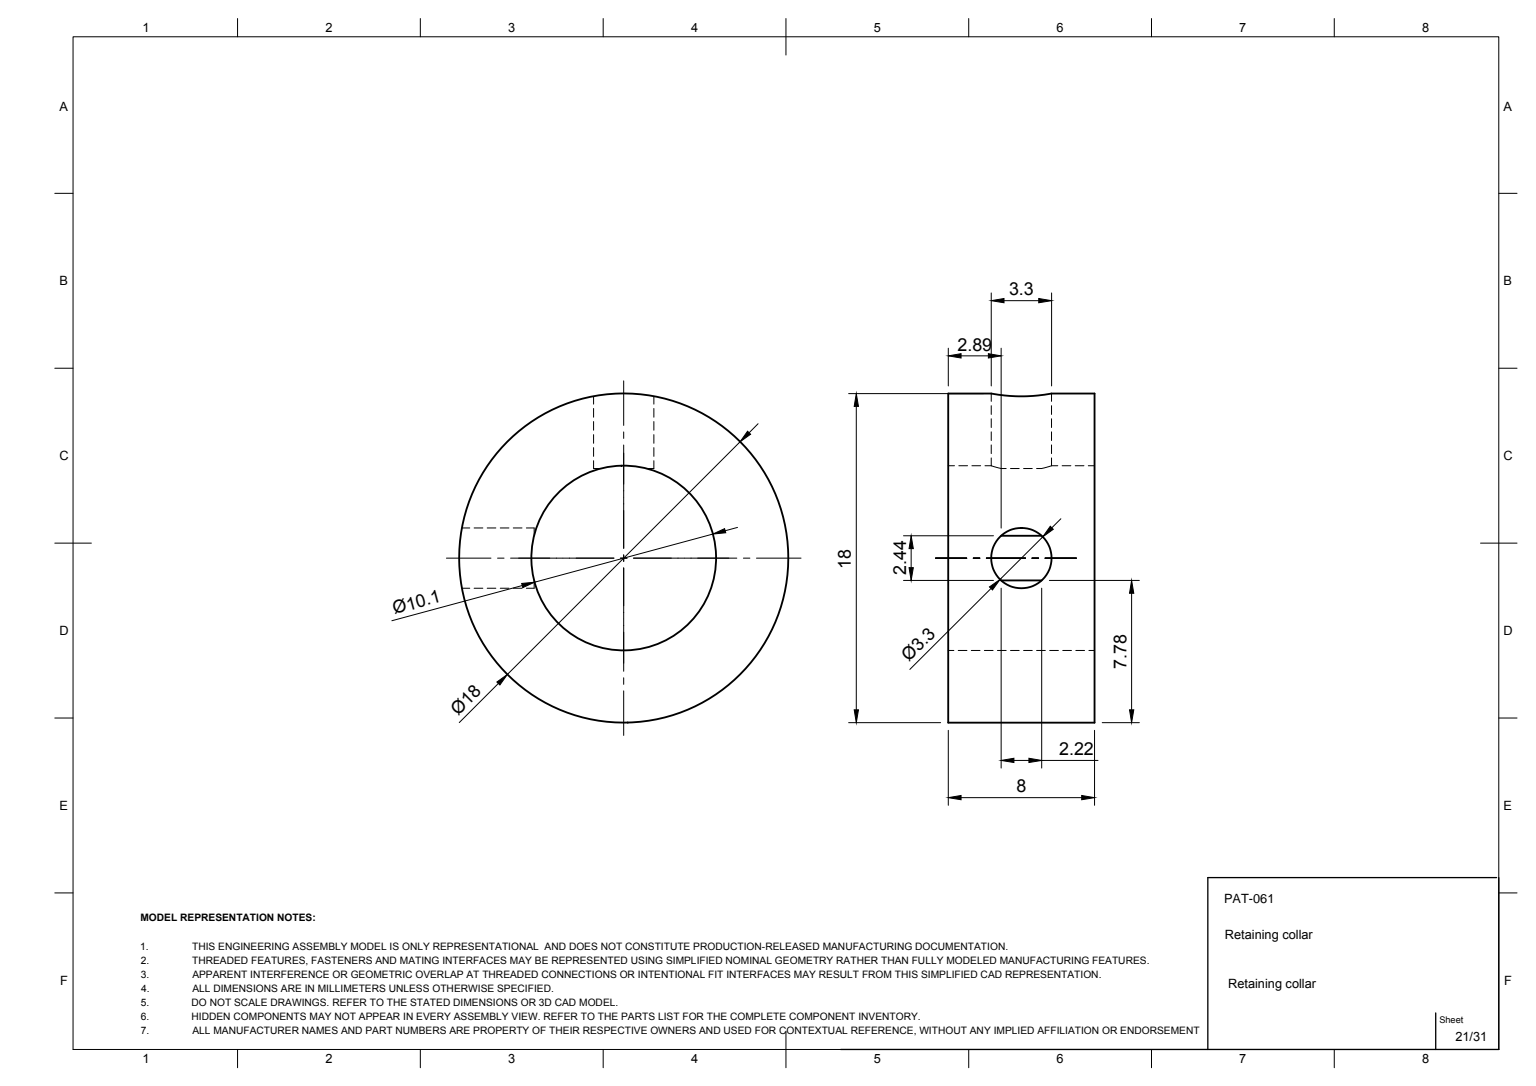
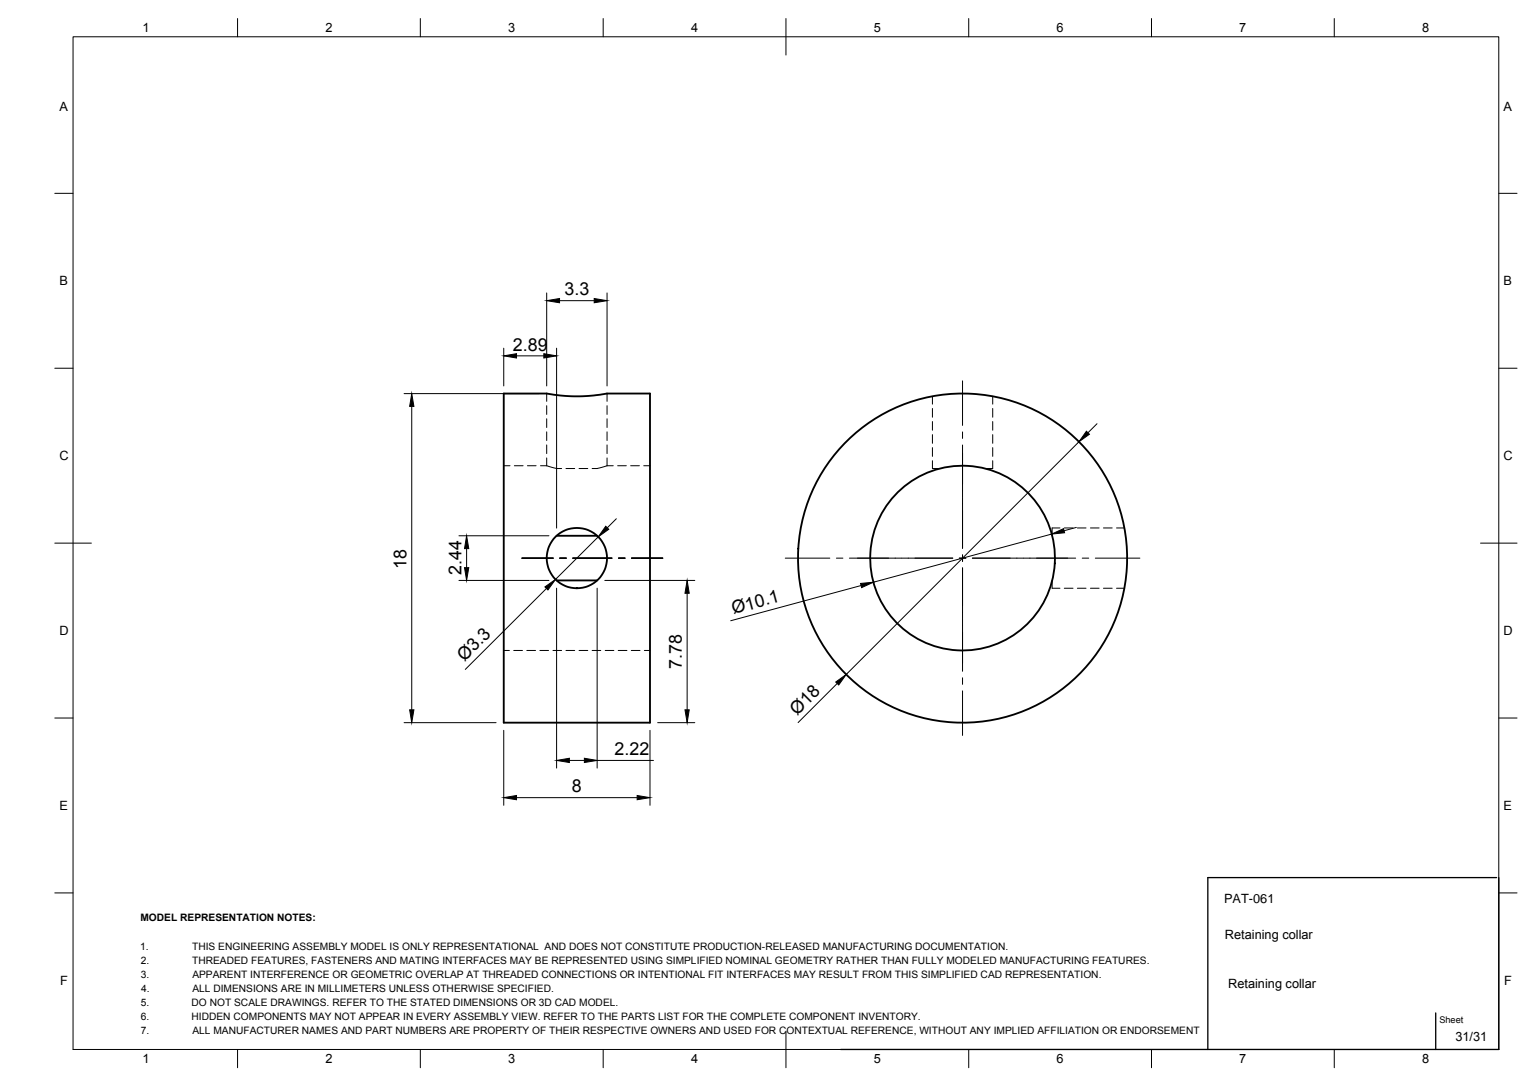
ISO-10303-21;
HEADER;
/* Generated by software containing ST-Developer
 * from STEP Tools, Inc. (www.steptools.com) 
 */

FILE_DESCRIPTION(
/* description */ ('Compact intermittent indexer'),
/* implementation_level */ '2;1');

FILE_NAME(
/* name */ 'Retaining collar.step',
/* time_stamp */ '2026-10-29T16:32:17-07:00',
/* author */ (''),
/* organization */ (''),
/* preprocessor_version */ 'ST-DEVELOPER v20.2',
/* originating_system */ 'Autodesk Translation Framework v15.17.0.0',
/* authorisation */ '');

FILE_SCHEMA (('AUTOMOTIVE_DESIGN { 1 0 10303 214 3 1 1 }'));
ENDSEC;

DATA;
#10=MECHANICAL_DESIGN_GEOMETRIC_PRESENTATION_REPRESENTATION('',(#278),#10837);
#222=SHAPE_REPRESENTATION_RELATIONSHIP('SRR','None',#10958,#246);
#246=ADVANCED_BREP_SHAPE_REPRESENTATION('',(#309),#10825);
#278=STYLED_ITEM('',(#11180),#309);
#309=MANIFOLD_SOLID_BREP('Body1',#5651);
#339=B_SPLINE_CURVE_WITH_KNOTS('',3,(#9829,#9830,#9831,#9832,#9833,#9834,
#9835,#9836,#9837,#9838,#9839,#9840,#9841,#9842,#9843,#9844,#9845,#9846,
#9847,#9848,#9849,#9850,#9851,#9852,#9853,#9854,#9855,#9856,#9857,#9858,
#9859,#9860,#9861,#9862),.UNSPECIFIED.,.T.,.F.,(4,2,2,2,2,2,2,2,2,2,2,2,
2,2,2,2,4),(0.,0.0623062782223143,0.124612556444629,0.186916384615149,0.249220212785669,
0.31152404095619,0.37382786912671,0.436134147349024,0.498440425571339,0.560746703793653,
0.623052982015967,0.685356810186488,0.747660638357008,0.809964466527529,
0.872268294698049,0.934574572920363,0.996880851142677),.UNSPECIFIED.);
#340=B_SPLINE_CURVE_WITH_KNOTS('',3,(#9865,#9866,#9867,#9868,#9869,#9870,
#9871,#9872,#9873,#9874,#9875,#9876,#9877,#9878),.UNSPECIFIED.,.F.,.F.,
(4,2,2,2,2,2,4),(0.618551524396292,0.626563103102765,0.689203386094988,
0.751843669087211,0.814483952079434,0.877124235071657,0.88513581377813),
 .UNSPECIFIED.);
#341=B_SPLINE_CURVE_WITH_KNOTS('',3,(#9881,#9882,#9883,#9884,#9885,#9886,
#9887,#9888,#9889,#9890,#9891,#9892,#9893,#9894),.UNSPECIFIED.,.F.,.F.,
(4,2,2,2,2,2,4),(0.117322411671485,0.125333990377958,0.187974273370181,
0.250614556362404,0.313254839354627,0.37589512234685,0.383906701053323),
 .UNSPECIFIED.);
#342=B_SPLINE_CURVE_WITH_KNOTS('',3,(#9905,#9906,#9907,#9908,#9909,#9910,
#9911,#9912,#9913,#9914),.UNSPECIFIED.,.F.,.F.,(4,2,2,2,4),(0.,0.0623062782223142,
0.124612556444628,0.186916384615149,0.249220212785669),.UNSPECIFIED.);
#343=B_SPLINE_CURVE_WITH_KNOTS('',3,(#9916,#9917,#9918,#9919,#9920,#9921,
#9922,#9923,#9924,#9925),.UNSPECIFIED.,.F.,.F.,(4,2,2,2,4),(0.747660638357008,
0.809964466527529,0.872268294698049,0.934574572920363,0.996880851142677),
 .UNSPECIFIED.);
#344=B_SPLINE_CURVE_WITH_KNOTS('',3,(#9926,#9927,#9928,#9929,#9930,#9931,
#9932,#9933,#9934,#9935,#9936,#9937,#9938,#9939,#9940,#9941,#9942,#9943),
 .UNSPECIFIED.,.F.,.F.,(4,2,2,2,2,2,2,2,4),(0.249220212785669,0.31152404095619,
0.37382786912671,0.436134147349024,0.498440425571339,0.560746703793653,
0.623052982015967,0.685356810186488,0.747660638357008),.UNSPECIFIED.);
#345=B_SPLINE_CURVE_WITH_KNOTS('',3,(#9947,#9948,#9949,#9950,#9951,#9952,
#9953,#9954),.UNSPECIFIED.,.F.,.F.,(4,2,2,4),(0.618551524396292,0.626563103102765,
0.689203386094988,0.751843669087211),.UNSPECIFIED.);
#346=B_SPLINE_CURVE_WITH_KNOTS('',3,(#9958,#9959,#9960,#9961,#9962,#9963,
#9964,#9965),.UNSPECIFIED.,.F.,.F.,(4,2,2,4),(0.250614556362404,0.313254839354627,
0.37589512234685,0.383906701053323),.UNSPECIFIED.);
#347=B_SPLINE_CURVE_WITH_KNOTS('',3,(#9966,#9967,#9968,#9969,#9970,#9971,
#9972,#9973),.UNSPECIFIED.,.F.,.F.,(4,2,2,4),(0.117322411671484,0.125333990377958,
0.187974273370181,0.250614556362404),.UNSPECIFIED.);
#348=B_SPLINE_CURVE_WITH_KNOTS('',3,(#9974,#9975,#9976,#9977,#9978,#9979,
#9980,#9981),.UNSPECIFIED.,.F.,.F.,(4,2,2,4),(0.751843669087211,0.814483952079434,
0.877124235071657,0.885135813778131),.UNSPECIFIED.);
#440=FACE_BOUND('',#1274,.T.);
#441=FACE_BOUND('',#1276,.T.);
#442=FACE_BOUND('',#1278,.T.);
#443=FACE_BOUND('',#1280,.T.);
#569=PLANE('',#6369);
#570=PLANE('',#6374);
#571=PLANE('',#6375);
#572=PLANE('',#6379);
#573=PLANE('',#6386);
#574=PLANE('',#6387);
#852=FACE_OUTER_BOUND('',#1267,.T.);
#853=FACE_OUTER_BOUND('',#1268,.T.);
#854=FACE_OUTER_BOUND('',#1269,.T.);
#855=FACE_OUTER_BOUND('',#1270,.T.);
#856=FACE_OUTER_BOUND('',#1271,.T.);
#857=FACE_OUTER_BOUND('',#1272,.T.);
#858=FACE_OUTER_BOUND('',#1273,.T.);
#859=FACE_OUTER_BOUND('',#1275,.T.);
#860=FACE_OUTER_BOUND('',#1277,.T.);
#861=FACE_OUTER_BOUND('',#1279,.T.);
#1267=EDGE_LOOP('',(#4530,#4531,#4532));
#1268=EDGE_LOOP('',(#4533,#4534,#4535,#4536,#4537,#4538,#4539,#4540));
#1269=EDGE_LOOP('',(#4541,#4542));
#1270=EDGE_LOOP('',(#4543,#4544));
#1271=EDGE_LOOP('',(#4545,#4546,#4547,#4548,#4549,#4550,#4551,#4552,#4553,
#4554,#4555));
#1272=EDGE_LOOP('',(#4556,#4557));
#1273=EDGE_LOOP('',(#4558,#4559,#4560,#4561,#4562,#4563,#4564,#4565,#4566,
#4567,#4568,#4569));
#1274=EDGE_LOOP('',(#4570,#4571,#4572,#4573));
#1275=EDGE_LOOP('',(#4574,#4575,#4576,#4577,#4578,#4579,#4580,#4581,#4582));
#1276=EDGE_LOOP('',(#4583));
#1277=EDGE_LOOP('',(#4584));
#1278=EDGE_LOOP('',(#4585));
#1279=EDGE_LOOP('',(#4586));
#1280=EDGE_LOOP('',(#4587));
#1605=LINE('',#9823,#1963);
#1606=LINE('',#9863,#1964);
#1607=LINE('',#9896,#1965);
#1608=LINE('',#9900,#1966);
#1609=LINE('',#9945,#1967);
#1610=LINE('',#9983,#1968);
#1611=LINE('',#9987,#1969);
#1612=LINE('',#9989,#1970);
#1613=LINE('',#9994,#1971);
#1614=LINE('',#9996,#1972);
#1963=VECTOR('',#7723,1.);
#1964=VECTOR('',#7730,0.165);
#1965=VECTOR('',#7735,1.);
#1966=VECTOR('',#7738,1.);
#1967=VECTOR('',#7743,0.165);
#1968=VECTOR('',#7748,1.);
#1969=VECTOR('',#7753,0.505);
#1970=VECTOR('',#7754,0.505);
#1971=VECTOR('',#7761,0.9);
#1972=VECTOR('',#7762,0.9);
#2366=CIRCLE('',#6370,0.165);
#2367=CIRCLE('',#6371,0.165);
#2368=CIRCLE('',#6373,0.165);
#2369=CIRCLE('',#6376,0.165);
#2370=CIRCLE('',#6378,0.165);
#2371=CIRCLE('',#6381,0.505);
#2372=CIRCLE('',#6382,0.505);
#2373=CIRCLE('',#6384,0.9);
#2374=CIRCLE('',#6385,0.9);
#2764=VERTEX_POINT('',#9821);
#2765=VERTEX_POINT('',#9822);
#2766=VERTEX_POINT('',#9824);
#2767=VERTEX_POINT('',#9828);
#2768=VERTEX_POINT('',#9864);
#2769=VERTEX_POINT('',#9879);
#2770=VERTEX_POINT('',#9898);
#2771=VERTEX_POINT('',#9899);
#2772=VERTEX_POINT('',#9903);
#2773=VERTEX_POINT('',#9904);
#2774=VERTEX_POINT('',#9915);
#2775=VERTEX_POINT('',#9944);
#2776=VERTEX_POINT('',#9946);
#2777=VERTEX_POINT('',#9955);
#2778=VERTEX_POINT('',#9957);
#2779=VERTEX_POINT('',#9985);
#2780=VERTEX_POINT('',#9988);
#2781=VERTEX_POINT('',#9992);
#2782=VERTEX_POINT('',#9995);
#3387=EDGE_CURVE('',#2764,#2765,#1605,.T.);
#3388=EDGE_CURVE('',#2766,#2764,#2366,.T.);
#3389=EDGE_CURVE('',#2765,#2766,#2367,.T.);
#3390=EDGE_CURVE('',#2767,#2767,#339,.T.);
#3391=EDGE_CURVE('',#2767,#2766,#1606,.T.);
#3392=EDGE_CURVE('',#2768,#2764,#340,.T.);
#3393=EDGE_CURVE('',#2768,#2769,#2368,.T.);
#3394=EDGE_CURVE('',#2765,#2769,#341,.T.);
#3395=EDGE_CURVE('',#2769,#2768,#1607,.T.);
#3396=EDGE_CURVE('',#2770,#2771,#1608,.T.);
#3397=EDGE_CURVE('',#2771,#2770,#2369,.T.);
#3398=EDGE_CURVE('',#2772,#2773,#342,.T.);
#3399=EDGE_CURVE('',#2774,#2772,#343,.T.);
#3400=EDGE_CURVE('',#2773,#2774,#344,.T.);
#3401=EDGE_CURVE('',#2773,#2775,#1609,.T.);
#3402=EDGE_CURVE('',#2776,#2775,#345,.T.);
#3403=EDGE_CURVE('',#2776,#2777,#2370,.T.);
#3404=EDGE_CURVE('',#2778,#2777,#346,.T.);
#3405=EDGE_CURVE('',#2771,#2778,#347,.T.);
#3406=EDGE_CURVE('',#2775,#2770,#348,.T.);
#3407=EDGE_CURVE('',#2777,#2776,#1610,.T.);
#3408=EDGE_CURVE('',#2779,#2779,#2371,.T.);
#3409=EDGE_CURVE('',#2779,#2775,#1611,.T.);
#3410=EDGE_CURVE('',#2778,#2780,#1612,.T.);
#3411=EDGE_CURVE('',#2780,#2780,#2372,.T.);
#3412=EDGE_CURVE('',#2781,#2781,#2373,.T.);
#3413=EDGE_CURVE('',#2781,#2773,#1613,.T.);
#3414=EDGE_CURVE('',#2774,#2782,#1614,.T.);
#3415=EDGE_CURVE('',#2782,#2782,#2374,.T.);
#4530=ORIENTED_EDGE('',*,*,#3387,.F.);
#4531=ORIENTED_EDGE('',*,*,#3388,.F.);
#4532=ORIENTED_EDGE('',*,*,#3389,.F.);
#4533=ORIENTED_EDGE('',*,*,#3390,.F.);
#4534=ORIENTED_EDGE('',*,*,#3391,.T.);
#4535=ORIENTED_EDGE('',*,*,#3388,.T.);
#4536=ORIENTED_EDGE('',*,*,#3392,.F.);
#4537=ORIENTED_EDGE('',*,*,#3393,.T.);
#4538=ORIENTED_EDGE('',*,*,#3394,.F.);
#4539=ORIENTED_EDGE('',*,*,#3389,.T.);
#4540=ORIENTED_EDGE('',*,*,#3391,.F.);
#4541=ORIENTED_EDGE('',*,*,#3395,.F.);
#4542=ORIENTED_EDGE('',*,*,#3393,.F.);
#4543=ORIENTED_EDGE('',*,*,#3396,.F.);
#4544=ORIENTED_EDGE('',*,*,#3397,.F.);
#4545=ORIENTED_EDGE('',*,*,#3398,.F.);
#4546=ORIENTED_EDGE('',*,*,#3399,.F.);
#4547=ORIENTED_EDGE('',*,*,#3400,.F.);
#4548=ORIENTED_EDGE('',*,*,#3401,.T.);
#4549=ORIENTED_EDGE('',*,*,#3402,.F.);
#4550=ORIENTED_EDGE('',*,*,#3403,.T.);
#4551=ORIENTED_EDGE('',*,*,#3404,.F.);
#4552=ORIENTED_EDGE('',*,*,#3405,.F.);
#4553=ORIENTED_EDGE('',*,*,#3397,.T.);
#4554=ORIENTED_EDGE('',*,*,#3406,.F.);
#4555=ORIENTED_EDGE('',*,*,#3401,.F.);
#4556=ORIENTED_EDGE('',*,*,#3407,.F.);
#4557=ORIENTED_EDGE('',*,*,#3403,.F.);
#4558=ORIENTED_EDGE('',*,*,#3408,.F.);
#4559=ORIENTED_EDGE('',*,*,#3409,.T.);
#4560=ORIENTED_EDGE('',*,*,#3406,.T.);
#4561=ORIENTED_EDGE('',*,*,#3396,.T.);
#4562=ORIENTED_EDGE('',*,*,#3405,.T.);
#4563=ORIENTED_EDGE('',*,*,#3410,.T.);
#4564=ORIENTED_EDGE('',*,*,#3411,.T.);
#4565=ORIENTED_EDGE('',*,*,#3410,.F.);
#4566=ORIENTED_EDGE('',*,*,#3404,.T.);
#4567=ORIENTED_EDGE('',*,*,#3407,.T.);
#4568=ORIENTED_EDGE('',*,*,#3402,.T.);
#4569=ORIENTED_EDGE('',*,*,#3409,.F.);
#4570=ORIENTED_EDGE('',*,*,#3394,.T.);
#4571=ORIENTED_EDGE('',*,*,#3395,.T.);
#4572=ORIENTED_EDGE('',*,*,#3392,.T.);
#4573=ORIENTED_EDGE('',*,*,#3387,.T.);
#4574=ORIENTED_EDGE('',*,*,#3412,.F.);
#4575=ORIENTED_EDGE('',*,*,#3413,.T.);
#4576=ORIENTED_EDGE('',*,*,#3400,.T.);
#4577=ORIENTED_EDGE('',*,*,#3414,.T.);
#4578=ORIENTED_EDGE('',*,*,#3415,.T.);
#4579=ORIENTED_EDGE('',*,*,#3414,.F.);
#4580=ORIENTED_EDGE('',*,*,#3399,.T.);
#4581=ORIENTED_EDGE('',*,*,#3398,.T.);
#4582=ORIENTED_EDGE('',*,*,#3413,.F.);
#4583=ORIENTED_EDGE('',*,*,#3390,.T.);
#4584=ORIENTED_EDGE('',*,*,#3412,.T.);
#4585=ORIENTED_EDGE('',*,*,#3408,.T.);
#4586=ORIENTED_EDGE('',*,*,#3415,.F.);
#4587=ORIENTED_EDGE('',*,*,#3411,.F.);
#5248=CYLINDRICAL_SURFACE('',#6372,0.165);
#5249=CYLINDRICAL_SURFACE('',#6377,0.165);
#5250=CYLINDRICAL_SURFACE('',#6380,0.505);
#5251=CYLINDRICAL_SURFACE('',#6383,0.9);
#5495=ADVANCED_FACE('',(#852),#569,.F.);
#5496=ADVANCED_FACE('',(#853),#5248,.F.);
#5497=ADVANCED_FACE('',(#854),#570,.F.);
#5498=ADVANCED_FACE('',(#855),#571,.F.);
#5499=ADVANCED_FACE('',(#856),#5249,.F.);
#5500=ADVANCED_FACE('',(#857),#572,.F.);
#5501=ADVANCED_FACE('',(#858,#440),#5250,.F.);
#5502=ADVANCED_FACE('',(#859,#441),#5251,.T.);
#5503=ADVANCED_FACE('',(#860,#442),#573,.T.);
#5504=ADVANCED_FACE('',(#861,#443),#574,.F.);
#5651=CLOSED_SHELL('',(#5495,#5496,#5497,#5498,#5499,#5500,#5501,#5502,
#5503,#5504));
#6368=AXIS2_PLACEMENT_3D('',#9819,#7719,#7720);
#6369=AXIS2_PLACEMENT_3D('',#9820,#7721,#7722);
#6370=AXIS2_PLACEMENT_3D('',#9825,#7724,#7725);
#6371=AXIS2_PLACEMENT_3D('',#9826,#7726,#7727);
#6372=AXIS2_PLACEMENT_3D('',#9827,#7728,#7729);
#6373=AXIS2_PLACEMENT_3D('',#9880,#7731,#7732);
#6374=AXIS2_PLACEMENT_3D('',#9895,#7733,#7734);
#6375=AXIS2_PLACEMENT_3D('',#9897,#7736,#7737);
#6376=AXIS2_PLACEMENT_3D('',#9901,#7739,#7740);
#6377=AXIS2_PLACEMENT_3D('',#9902,#7741,#7742);
#6378=AXIS2_PLACEMENT_3D('',#9956,#7744,#7745);
#6379=AXIS2_PLACEMENT_3D('',#9982,#7746,#7747);
#6380=AXIS2_PLACEMENT_3D('',#9984,#7749,#7750);
#6381=AXIS2_PLACEMENT_3D('',#9986,#7751,#7752);
#6382=AXIS2_PLACEMENT_3D('',#9990,#7755,#7756);
#6383=AXIS2_PLACEMENT_3D('',#9991,#7757,#7758);
#6384=AXIS2_PLACEMENT_3D('',#9993,#7759,#7760);
#6385=AXIS2_PLACEMENT_3D('',#9997,#7763,#7764);
#6386=AXIS2_PLACEMENT_3D('',#9998,#7765,#7766);
#6387=AXIS2_PLACEMENT_3D('',#9999,#7767,#7768);
#7719=DIRECTION('axis',(0.,0.,1.));
#7720=DIRECTION('refdir',(1.,0.,0.));
#7721=DIRECTION('center_axis',(0.,1.,0.));
#7722=DIRECTION('ref_axis',(1.,0.,0.));
#7723=DIRECTION('',(0.,0.,-1.));
#7724=DIRECTION('center_axis',(0.,1.,0.));
#7725=DIRECTION('ref_axis',(1.,0.,0.));
#7726=DIRECTION('center_axis',(0.,1.,0.));
#7727=DIRECTION('ref_axis',(1.,0.,0.));
#7728=DIRECTION('center_axis',(0.,1.,0.));
#7729=DIRECTION('ref_axis',(1.,0.,0.));
#7730=DIRECTION('',(0.,1.,0.));
#7731=DIRECTION('center_axis',(0.,1.,0.));
#7732=DIRECTION('ref_axis',(1.,0.,0.));
#7733=DIRECTION('center_axis',(0.,1.,0.));
#7734=DIRECTION('ref_axis',(1.,0.,0.));
#7735=DIRECTION('',(0.,0.,1.));
#7736=DIRECTION('center_axis',(1.,0.,0.));
#7737=DIRECTION('ref_axis',(0.,0.,-1.));
#7738=DIRECTION('',(0.,0.,-1.));
#7739=DIRECTION('center_axis',(1.,0.,0.));
#7740=DIRECTION('ref_axis',(0.,0.,-1.));
#7741=DIRECTION('center_axis',(1.,0.,0.));
#7742=DIRECTION('ref_axis',(0.,0.,-1.));
#7743=DIRECTION('',(1.,0.,0.));
#7744=DIRECTION('center_axis',(1.,0.,0.));
#7745=DIRECTION('ref_axis',(0.,0.,-1.));
#7746=DIRECTION('center_axis',(1.,0.,0.));
#7747=DIRECTION('ref_axis',(0.,0.,-1.));
#7748=DIRECTION('',(0.,0.,1.));
#7749=DIRECTION('center_axis',(0.,0.,1.));
#7750=DIRECTION('ref_axis',(1.,0.,0.));
#7751=DIRECTION('center_axis',(0.,0.,-1.));
#7752=DIRECTION('ref_axis',(1.,0.,0.));
#7753=DIRECTION('',(0.,0.,-1.));
#7754=DIRECTION('',(0.,0.,-1.));
#7755=DIRECTION('center_axis',(0.,0.,-1.));
#7756=DIRECTION('ref_axis',(1.,0.,0.));
#7757=DIRECTION('center_axis',(0.,0.,1.));
#7758=DIRECTION('ref_axis',(1.,0.,0.));
#7759=DIRECTION('center_axis',(0.,0.,1.));
#7760=DIRECTION('ref_axis',(1.,0.,0.));
#7761=DIRECTION('',(0.,0.,-1.));
#7762=DIRECTION('',(0.,0.,-1.));
#7763=DIRECTION('center_axis',(0.,0.,1.));
#7764=DIRECTION('ref_axis',(1.,0.,0.));
#7765=DIRECTION('center_axis',(0.,0.,1.));
#7766=DIRECTION('ref_axis',(1.,0.,0.));
#7767=DIRECTION('center_axis',(0.,0.,1.));
#7768=DIRECTION('ref_axis',(1.,0.,0.));
#9819=CARTESIAN_POINT('',(0.,0.,0.));
#9820=CARTESIAN_POINT('Origin',(0.,-0.49,1.4));
#9821=CARTESIAN_POINT('',(-0.122167917228706,-0.49,1.51090536506409));
#9822=CARTESIAN_POINT('',(-0.122167917228706,-0.49,1.28909463493591));
#9823=CARTESIAN_POINT('',(-0.122167917228706,-0.49,1.));
#9824=CARTESIAN_POINT('',(-0.165,-0.49,1.4));
#9825=CARTESIAN_POINT('Origin',(0.,-0.49,1.4));
#9826=CARTESIAN_POINT('Origin',(0.,-0.49,1.4));
#9827=CARTESIAN_POINT('Origin',(0.,-1.,1.4));
#9828=CARTESIAN_POINT('',(-0.165,-0.884745726183518,1.4));
#9829=CARTESIAN_POINT('Ctrl Pts',(-0.165,-0.884745726183518,1.4));
#9830=CARTESIAN_POINT('Ctrl Pts',(-0.165,-0.884745726183518,1.42076875940744));
#9831=CARTESIAN_POINT('Ctrl Pts',(-0.160839719007584,-0.885552759505264,
1.44288889507334));
#9832=CARTESIAN_POINT('Ctrl Pts',(-0.14398647021669,-0.888448648150043,
1.48352706263377));
#9833=CARTESIAN_POINT('Ctrl Pts',(-0.131295993814186,-0.890493604851638,
1.50204924397737));
#9834=CARTESIAN_POINT('Ctrl Pts',(-0.102049819008125,-0.89431723432394,
1.53129541878344));
#9835=CARTESIAN_POINT('Ctrl Pts',(-0.0835273920906823,-0.896347088899543,
1.54398634598358));
#9836=CARTESIAN_POINT('Ctrl Pts',(-0.0428883760934128,-0.899208271860583,
1.56083992183864));
#9837=CARTESIAN_POINT('Ctrl Pts',(-0.0207679427235068,-0.9,1.565));
#9838=CARTESIAN_POINT('Ctrl Pts',(0.0207679427235068,-0.9,1.565));
#9839=CARTESIAN_POINT('Ctrl Pts',(0.0428883760934127,-0.899208271860583,
1.56083992183864));
#9840=CARTESIAN_POINT('Ctrl Pts',(0.0835273920906823,-0.896347088899543,
1.54398634598358));
#9841=CARTESIAN_POINT('Ctrl Pts',(0.102049819008125,-0.89431723432394,1.53129541878344));
#9842=CARTESIAN_POINT('Ctrl Pts',(0.131295993814186,-0.890493604851638,
1.50204924397737));
#9843=CARTESIAN_POINT('Ctrl Pts',(0.14398647021669,-0.888448648150043,1.48352706263377));
#9844=CARTESIAN_POINT('Ctrl Pts',(0.160839719007584,-0.885552759505264,
1.44288889507334));
#9845=CARTESIAN_POINT('Ctrl Pts',(0.165,-0.884745726183518,1.42076875940744));
#9846=CARTESIAN_POINT('Ctrl Pts',(0.165,-0.884745726183518,1.37923124059256));
#9847=CARTESIAN_POINT('Ctrl Pts',(0.160839719007584,-0.885552759505264,
1.35711110492666));
#9848=CARTESIAN_POINT('Ctrl Pts',(0.14398647021669,-0.888448648150043,1.31647293736623));
#9849=CARTESIAN_POINT('Ctrl Pts',(0.131295993814186,-0.890493604851638,
1.29795075602263));
#9850=CARTESIAN_POINT('Ctrl Pts',(0.102049819008125,-0.89431723432394,1.26870458121656));
#9851=CARTESIAN_POINT('Ctrl Pts',(0.0835273920906823,-0.896347088899543,
1.25601365401642));
#9852=CARTESIAN_POINT('Ctrl Pts',(0.0428883760934127,-0.899208271860583,
1.23916007816136));
#9853=CARTESIAN_POINT('Ctrl Pts',(0.0207679427235068,-0.9,1.235));
#9854=CARTESIAN_POINT('Ctrl Pts',(-0.0207679427235067,-0.9,1.235));
#9855=CARTESIAN_POINT('Ctrl Pts',(-0.0428883760934127,-0.899208271860583,
1.23916007816136));
#9856=CARTESIAN_POINT('Ctrl Pts',(-0.0835273920906822,-0.896347088899543,
1.25601365401642));
#9857=CARTESIAN_POINT('Ctrl Pts',(-0.102049819008125,-0.89431723432394,
1.26870458121656));
#9858=CARTESIAN_POINT('Ctrl Pts',(-0.131295993814186,-0.890493604851638,
1.29795075602263));
#9859=CARTESIAN_POINT('Ctrl Pts',(-0.14398647021669,-0.888448648150043,
1.31647293736623));
#9860=CARTESIAN_POINT('Ctrl Pts',(-0.160839719007584,-0.885552759505264,
1.35711110492666));
#9861=CARTESIAN_POINT('Ctrl Pts',(-0.165,-0.884745726183518,1.37923124059256));
#9862=CARTESIAN_POINT('Ctrl Pts',(-0.165,-0.884745726183518,1.4));
#9863=CARTESIAN_POINT('',(-0.165,-1.,1.4));
#9864=CARTESIAN_POINT('',(0.122167917228706,-0.49,1.51090536506409));
#9865=CARTESIAN_POINT('Ctrl Pts',(0.122167917228706,-0.49,1.51090536506409));
#9866=CARTESIAN_POINT('Ctrl Pts',(0.120368913626296,-0.490448531679987,
1.51288705930464));
#9867=CARTESIAN_POINT('Ctrl Pts',(0.118534896565231,-0.490895245371684,
1.51481034122633));
#9868=CARTESIAN_POINT('Ctrl Pts',(0.102111993019358,-0.494795015531646,
1.5312332447722));
#9869=CARTESIAN_POINT('Ctrl Pts',(0.0836597150224318,-0.498442514607594,
1.54390845611142));
#9870=CARTESIAN_POINT('Ctrl Pts',(0.0430495960471595,-0.50357781976106,
1.56079590960766));
#9871=CARTESIAN_POINT('Ctrl Pts',(0.020880094330741,-0.505,1.565));
#9872=CARTESIAN_POINT('Ctrl Pts',(-0.020880094330741,-0.505,1.565));
#9873=CARTESIAN_POINT('Ctrl Pts',(-0.0430495960471594,-0.50357781976106,
1.56079590960766));
#9874=CARTESIAN_POINT('Ctrl Pts',(-0.0836597150224317,-0.498442514607594,
1.54390845611142));
#9875=CARTESIAN_POINT('Ctrl Pts',(-0.102111993019358,-0.494795015531646,
1.5312332447722));
#9876=CARTESIAN_POINT('Ctrl Pts',(-0.118534896565231,-0.490895245371684,
1.51481034122633));
#9877=CARTESIAN_POINT('Ctrl Pts',(-0.120368913626296,-0.490448531679987,
1.51288705930464));
#9878=CARTESIAN_POINT('Ctrl Pts',(-0.122167917228706,-0.49,1.51090536506409));
#9879=CARTESIAN_POINT('',(0.122167917228706,-0.49,1.28909463493591));
#9880=CARTESIAN_POINT('Origin',(0.,-0.49,1.4));
#9881=CARTESIAN_POINT('Ctrl Pts',(-0.122167917228706,-0.49,1.28909463493591));
#9882=CARTESIAN_POINT('Ctrl Pts',(-0.120368913626296,-0.490448531679987,
1.28711294069536));
#9883=CARTESIAN_POINT('Ctrl Pts',(-0.118534896565231,-0.490895245371684,
1.28518965877367));
#9884=CARTESIAN_POINT('Ctrl Pts',(-0.102111993019358,-0.494795015531646,
1.2687667552278));
#9885=CARTESIAN_POINT('Ctrl Pts',(-0.0836597150224318,-0.498442514607594,
1.25609154388858));
#9886=CARTESIAN_POINT('Ctrl Pts',(-0.0430495960471595,-0.50357781976106,
1.23920409039234));
#9887=CARTESIAN_POINT('Ctrl Pts',(-0.020880094330741,-0.505,1.235));
#9888=CARTESIAN_POINT('Ctrl Pts',(0.020880094330741,-0.505,1.235));
#9889=CARTESIAN_POINT('Ctrl Pts',(0.0430495960471595,-0.50357781976106,
1.23920409039234));
#9890=CARTESIAN_POINT('Ctrl Pts',(0.0836597150224318,-0.498442514607594,
1.25609154388858));
#9891=CARTESIAN_POINT('Ctrl Pts',(0.102111993019358,-0.494795015531646,
1.2687667552278));
#9892=CARTESIAN_POINT('Ctrl Pts',(0.118534896565231,-0.490895245371684,
1.28518965877367));
#9893=CARTESIAN_POINT('Ctrl Pts',(0.120368913626296,-0.490448531679987,
1.28711294069536));
#9894=CARTESIAN_POINT('Ctrl Pts',(0.122167917228706,-0.49,1.28909463493591));
#9895=CARTESIAN_POINT('Origin',(0.,-0.49,1.4));
#9896=CARTESIAN_POINT('',(0.122167917228706,-0.49,1.));
#9897=CARTESIAN_POINT('Origin',(-0.49,0.,1.4));
#9898=CARTESIAN_POINT('',(-0.49,0.122167917228706,1.51090536506409));
#9899=CARTESIAN_POINT('',(-0.49,0.122167917228706,1.28909463493591));
#9900=CARTESIAN_POINT('',(-0.49,0.122167917228706,1.));
#9901=CARTESIAN_POINT('Origin',(-0.49,0.,1.4));
#9902=CARTESIAN_POINT('Origin',(-1.,0.,1.4));
#9903=CARTESIAN_POINT('',(-0.884745726183518,0.165,1.4));
#9904=CARTESIAN_POINT('',(-0.9,-2.02066721859313E-17,1.565));
#9905=CARTESIAN_POINT('Ctrl Pts',(-0.884745726183518,0.165,1.4));
#9906=CARTESIAN_POINT('Ctrl Pts',(-0.884745726183518,0.165,1.42076875940744));
#9907=CARTESIAN_POINT('Ctrl Pts',(-0.885552759505264,0.160839719007584,
1.44288889507334));
#9908=CARTESIAN_POINT('Ctrl Pts',(-0.888448648150043,0.14398647021669,1.48352706263377));
#9909=CARTESIAN_POINT('Ctrl Pts',(-0.890493604851638,0.131295993814186,
1.50204924397737));
#9910=CARTESIAN_POINT('Ctrl Pts',(-0.89431723432394,0.102049819008125,1.53129541878344));
#9911=CARTESIAN_POINT('Ctrl Pts',(-0.896347088899543,0.0835273920906824,
1.54398634598358));
#9912=CARTESIAN_POINT('Ctrl Pts',(-0.899208271860583,0.0428883760934128,
1.56083992183864));
#9913=CARTESIAN_POINT('Ctrl Pts',(-0.9,0.0207679427235068,1.565));
#9914=CARTESIAN_POINT('Ctrl Pts',(-0.9,2.77555756156289E-17,1.565));
#9915=CARTESIAN_POINT('',(-0.9,-8.63341285292134E-17,1.235));
#9916=CARTESIAN_POINT('Ctrl Pts',(-0.9,-6.24500451351651E-17,1.235));
#9917=CARTESIAN_POINT('Ctrl Pts',(-0.9,0.0207679427235068,1.235));
#9918=CARTESIAN_POINT('Ctrl Pts',(-0.899208271860583,0.0428883760934128,
1.23916007816136));
#9919=CARTESIAN_POINT('Ctrl Pts',(-0.896347088899543,0.0835273920906824,
1.25601365401642));
#9920=CARTESIAN_POINT('Ctrl Pts',(-0.89431723432394,0.102049819008125,1.26870458121656));
#9921=CARTESIAN_POINT('Ctrl Pts',(-0.890493604851638,0.131295993814186,
1.29795075602263));
#9922=CARTESIAN_POINT('Ctrl Pts',(-0.888448648150043,0.143986470216691,
1.31647293736623));
#9923=CARTESIAN_POINT('Ctrl Pts',(-0.885552759505264,0.160839719007584,
1.35711110492666));
#9924=CARTESIAN_POINT('Ctrl Pts',(-0.884745726183518,0.165,1.37923124059256));
#9925=CARTESIAN_POINT('Ctrl Pts',(-0.884745726183518,0.165,1.4));
#9926=CARTESIAN_POINT('Ctrl Pts',(-0.9,4.16333634234434E-17,1.565));
#9927=CARTESIAN_POINT('Ctrl Pts',(-0.9,-0.0207679427235068,1.565));
#9928=CARTESIAN_POINT('Ctrl Pts',(-0.899208271860583,-0.0428883760934127,
1.56083992183864));
#9929=CARTESIAN_POINT('Ctrl Pts',(-0.896347088899543,-0.0835273920906824,
1.54398634598358));
#9930=CARTESIAN_POINT('Ctrl Pts',(-0.89431723432394,-0.102049819008125,
1.53129541878344));
#9931=CARTESIAN_POINT('Ctrl Pts',(-0.890493604851638,-0.131295993814186,
1.50204924397737));
#9932=CARTESIAN_POINT('Ctrl Pts',(-0.888448648150043,-0.143986470216691,
1.48352706263377));
#9933=CARTESIAN_POINT('Ctrl Pts',(-0.885552759505264,-0.160839719007584,
1.44288889507334));
#9934=CARTESIAN_POINT('Ctrl Pts',(-0.884745726183518,-0.165,1.42076875940744));
#9935=CARTESIAN_POINT('Ctrl Pts',(-0.884745726183518,-0.165,1.37923124059256));
#9936=CARTESIAN_POINT('Ctrl Pts',(-0.885552759505264,-0.160839719007584,
1.35711110492666));
#9937=CARTESIAN_POINT('Ctrl Pts',(-0.888448648150043,-0.14398647021669,
1.31647293736623));
#9938=CARTESIAN_POINT('Ctrl Pts',(-0.890493604851638,-0.131295993814186,
1.29795075602263));
#9939=CARTESIAN_POINT('Ctrl Pts',(-0.89431723432394,-0.102049819008125,
1.26870458121656));
#9940=CARTESIAN_POINT('Ctrl Pts',(-0.896347088899543,-0.0835273920906825,
1.25601365401642));
#9941=CARTESIAN_POINT('Ctrl Pts',(-0.899208271860583,-0.0428883760934129,
1.23916007816136));
#9942=CARTESIAN_POINT('Ctrl Pts',(-0.9,-0.0207679427235069,1.235));
#9943=CARTESIAN_POINT('Ctrl Pts',(-0.9,-4.85722573273506E-17,1.235));
#9944=CARTESIAN_POINT('',(-0.505,-2.74505708527337E-17,1.565));
#9945=CARTESIAN_POINT('',(-1.,-2.02066721859313E-17,1.565));
#9946=CARTESIAN_POINT('',(-0.49,-0.122167917228706,1.51090536506409));
#9947=CARTESIAN_POINT('Ctrl Pts',(-0.49,-0.122167917228706,1.51090536506409));
#9948=CARTESIAN_POINT('Ctrl Pts',(-0.490448531679987,-0.120368913626296,
1.51288705930464));
#9949=CARTESIAN_POINT('Ctrl Pts',(-0.490895245371684,-0.118534896565231,
1.51481034122633));
#9950=CARTESIAN_POINT('Ctrl Pts',(-0.494795015531646,-0.102111993019358,
1.5312332447722));
#9951=CARTESIAN_POINT('Ctrl Pts',(-0.498442514607594,-0.0836597150224318,
1.54390845611142));
#9952=CARTESIAN_POINT('Ctrl Pts',(-0.50357781976106,-0.0430495960471595,
1.56079590960766));
#9953=CARTESIAN_POINT('Ctrl Pts',(-0.505,-0.020880094330741,1.565));
#9954=CARTESIAN_POINT('Ctrl Pts',(-0.505,0.,1.565));
#9955=CARTESIAN_POINT('',(-0.49,-0.122167917228706,1.28909463493591));
#9956=CARTESIAN_POINT('Origin',(-0.49,0.,1.4));
#9957=CARTESIAN_POINT('',(-0.505,-2.05139908226098E-17,1.235));
#9958=CARTESIAN_POINT('Ctrl Pts',(-0.505,2.77555756156289E-17,1.235));
#9959=CARTESIAN_POINT('Ctrl Pts',(-0.505,-0.020880094330741,1.235));
#9960=CARTESIAN_POINT('Ctrl Pts',(-0.50357781976106,-0.0430495960471594,
1.23920409039234));
#9961=CARTESIAN_POINT('Ctrl Pts',(-0.498442514607595,-0.0836597150224317,
1.25609154388858));
#9962=CARTESIAN_POINT('Ctrl Pts',(-0.494795015531646,-0.102111993019358,
1.2687667552278));
#9963=CARTESIAN_POINT('Ctrl Pts',(-0.490895245371684,-0.118534896565231,
1.28518965877367));
#9964=CARTESIAN_POINT('Ctrl Pts',(-0.490448531679987,-0.120368913626296,
1.28711294069536));
#9965=CARTESIAN_POINT('Ctrl Pts',(-0.49,-0.122167917228706,1.28909463493591));
#9966=CARTESIAN_POINT('Ctrl Pts',(-0.49,0.122167917228706,1.28909463493591));
#9967=CARTESIAN_POINT('Ctrl Pts',(-0.490448531679987,0.120368913626296,
1.28711294069536));
#9968=CARTESIAN_POINT('Ctrl Pts',(-0.490895245371684,0.118534896565231,
1.28518965877367));
#9969=CARTESIAN_POINT('Ctrl Pts',(-0.494795015531646,0.102111993019358,
1.2687667552278));
#9970=CARTESIAN_POINT('Ctrl Pts',(-0.498442514607594,0.0836597150224318,
1.25609154388858));
#9971=CARTESIAN_POINT('Ctrl Pts',(-0.50357781976106,0.0430495960471595,
1.23920409039234));
#9972=CARTESIAN_POINT('Ctrl Pts',(-0.505,0.020880094330741,1.235));
#9973=CARTESIAN_POINT('Ctrl Pts',(-0.505,-6.93889390390723E-18,1.235));
#9974=CARTESIAN_POINT('Ctrl Pts',(-0.505,-2.77555756156289E-17,1.565));
#9975=CARTESIAN_POINT('Ctrl Pts',(-0.505,0.020880094330741,1.565));
#9976=CARTESIAN_POINT('Ctrl Pts',(-0.50357781976106,0.0430495960471595,
1.56079590960766));
#9977=CARTESIAN_POINT('Ctrl Pts',(-0.498442514607594,0.0836597150224318,
1.54390845611142));
#9978=CARTESIAN_POINT('Ctrl Pts',(-0.494795015531646,0.102111993019358,
1.5312332447722));
#9979=CARTESIAN_POINT('Ctrl Pts',(-0.490895245371684,0.118534896565231,
1.51481034122633));
#9980=CARTESIAN_POINT('Ctrl Pts',(-0.490448531679987,0.120368913626296,
1.51288705930464));
#9981=CARTESIAN_POINT('Ctrl Pts',(-0.49,0.122167917228706,1.51090536506409));
#9982=CARTESIAN_POINT('Origin',(-0.49,0.,1.4));
#9983=CARTESIAN_POINT('',(-0.49,-0.122167917228706,1.));
#9984=CARTESIAN_POINT('Origin',(0.,0.,1.));
#9985=CARTESIAN_POINT('',(-0.505,-6.18446633569413E-17,1.8));
#9986=CARTESIAN_POINT('Origin',(0.,0.,1.8));
#9987=CARTESIAN_POINT('',(-0.505,-6.18446633569413E-17,1.));
#9988=CARTESIAN_POINT('',(-0.505,-6.18446633569413E-17,1.));
#9989=CARTESIAN_POINT('',(-0.505,-6.18446633569413E-17,1.));
#9990=CARTESIAN_POINT('Origin',(0.,0.,1.));
#9991=CARTESIAN_POINT('Origin',(0.,0.,1.));
#9992=CARTESIAN_POINT('',(-0.9,-1.10218211923262E-16,1.8));
#9993=CARTESIAN_POINT('Origin',(0.,0.,1.8));
#9994=CARTESIAN_POINT('',(-0.9,-1.10218211923262E-16,1.));
#9995=CARTESIAN_POINT('',(-0.9,-1.10218211923262E-16,1.));
#9996=CARTESIAN_POINT('',(-0.9,-1.10218211923262E-16,1.));
#9997=CARTESIAN_POINT('Origin',(0.,0.,1.));
#9998=CARTESIAN_POINT('Origin',(0.,0.,1.8));
#9999=CARTESIAN_POINT('Origin',(0.,0.,1.));
#10795=UNCERTAINTY_MEASURE_WITH_UNIT(LENGTH_MEASURE(0.001),#10838,
'DISTANCE_ACCURACY_VALUE',
'Maximum model space distance between geometric entities at asserted c
onnectivities');
#10807=UNCERTAINTY_MEASURE_WITH_UNIT(LENGTH_MEASURE(0.001),#10838,
'DISTANCE_ACCURACY_VALUE',
'Maximum model space distance between geometric entities at asserted c
onnectivities');
#10825=(
GEOMETRIC_REPRESENTATION_CONTEXT(3)
GLOBAL_UNCERTAINTY_ASSIGNED_CONTEXT((#10795))
GLOBAL_UNIT_ASSIGNED_CONTEXT((#10838,#10840,#10841))
REPRESENTATION_CONTEXT('','3D')
);
#10837=(
GEOMETRIC_REPRESENTATION_CONTEXT(3)
GLOBAL_UNCERTAINTY_ASSIGNED_CONTEXT((#10807))
GLOBAL_UNIT_ASSIGNED_CONTEXT((#10838,#10840,#10841))
REPRESENTATION_CONTEXT('','3D')
);
#10838=(
LENGTH_UNIT()
NAMED_UNIT(*)
SI_UNIT(.CENTI.,.METRE.)
);
#10840=(
NAMED_UNIT(*)
PLANE_ANGLE_UNIT()
SI_UNIT($,.RADIAN.)
);
#10841=(
NAMED_UNIT(*)
SI_UNIT($,.STERADIAN.)
SOLID_ANGLE_UNIT()
);
#10859=SHAPE_DEFINITION_REPRESENTATION(#10893,#10958);
#10893=PRODUCT_DEFINITION_SHAPE('',$,#10988);
#10958=SHAPE_REPRESENTATION('',(#6368),#10825);
#10970=PRODUCT_DEFINITION_CONTEXT('part definition',#11059,'design');
#10988=PRODUCT_DEFINITION('Retaining collar','Retaining collar',#11017,
#10970);
#11017=PRODUCT_DEFINITION_FORMATION('',$,#11078);
#11059=APPLICATION_CONTEXT(
'Core Data for Automotive Mechanical Design Process');
#11060=PRODUCT_CONTEXT('part definition',#11059,'mechanical');
#11078=PRODUCT('Retaining collar','Retaining collar','Retaining collar',
(#11060));
#11174=COLOUR_RGB('Off White',0.89,0.88,0.83);
#11175=FILL_AREA_STYLE_COLOUR('',#11174);
#11176=FILL_AREA_STYLE('',(#11175));
#11177=SURFACE_STYLE_FILL_AREA(#11176);
#11178=SURFACE_SIDE_STYLE('',(#11177));
#11179=SURFACE_STYLE_USAGE(.BOTH.,#11178);
#11180=PRESENTATION_STYLE_ASSIGNMENT((#11179));
ENDSEC;
END-ISO-10303-21;
